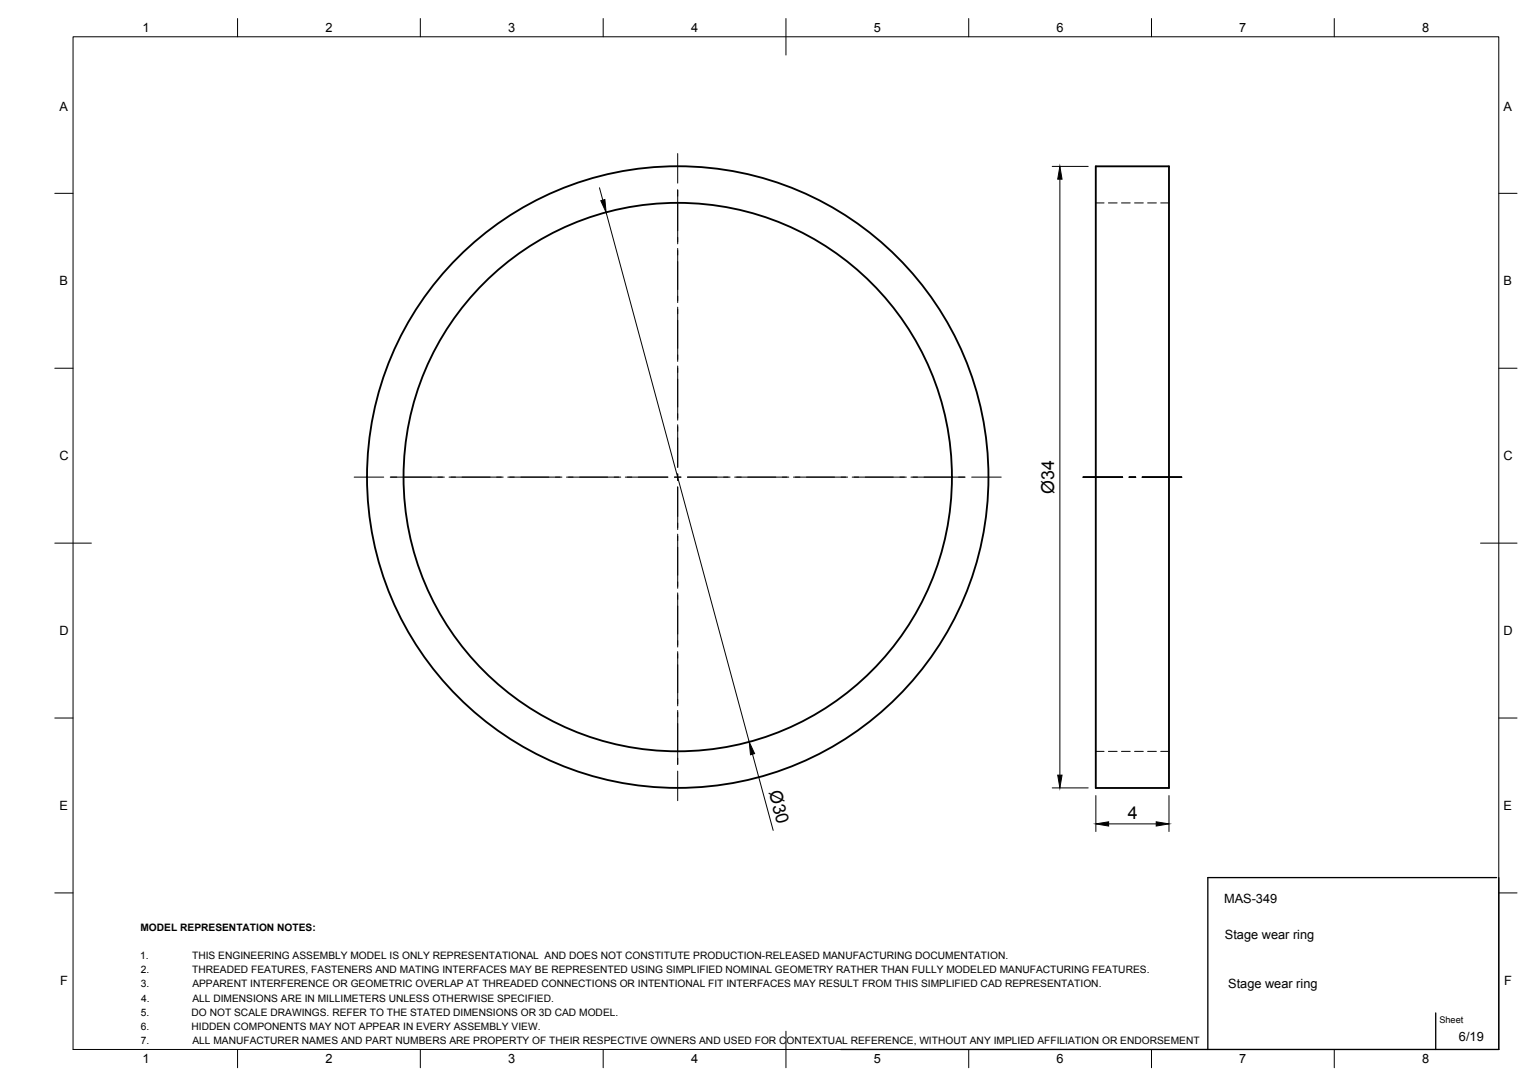
ISO-10303-21;
HEADER;
/* Generated by software containing ST-Developer
 * from STEP Tools, Inc. (www.steptools.com) 
 */

FILE_DESCRIPTION(
/* description */ ('Independent two-stage semi-open centrifugal-pump CAD. Shared impeller
s, open-machinable return casings, removable diaphragms, bronze wear/j
ournal rings, volume-preserving seal instances, retained keyed shaft, 
opposed mechanical face rings and partly threaded tie hardware. Native
 shaft rotation. Geometric topology/clearance only; flow/head/efficien
cy, pressure, cavitation, balance, preload, face loading and secondary
 seal fits/bonds, material/thermal/tolerance selection and life unassi
gned. External drive, coupling, anchors and piping bolts omitted.'),
/* implementation_level */ '2;1');

FILE_NAME(
/* name */ 'Stage wear ring.step',
/* time_stamp */ '2026-11-08T18:06:32-08:00',
/* author */ (''),
/* organization */ (''),
/* preprocessor_version */ 'ST-DEVELOPER v20.2',
/* originating_system */ 'Autodesk Translation Framework v15.17.0.0',
/* authorisation */ '');

FILE_SCHEMA (('AUTOMOTIVE_DESIGN { 1 0 10303 214 3 1 1 }'));
ENDSEC;

DATA;
#10=MECHANICAL_DESIGN_GEOMETRIC_PRESENTATION_REPRESENTATION('',(#396),#16687);
#358=SHAPE_REPRESENTATION_RELATIONSHIP('SRR','None',#16767,#377);
#377=ADVANCED_BREP_SHAPE_REPRESENTATION('',(#415),#16671);
#396=STYLED_ITEM('',(#16871),#415);
#415=MANIFOLD_SOLID_BREP('Body1',#6115);
#475=FACE_BOUND('',#1186,.T.);
#476=FACE_BOUND('',#1188,.T.);
#612=PLANE('',#6560);
#613=PLANE('',#6561);
#792=FACE_OUTER_BOUND('',#1183,.T.);
#793=FACE_OUTER_BOUND('',#1184,.T.);
#794=FACE_OUTER_BOUND('',#1185,.T.);
#795=FACE_OUTER_BOUND('',#1187,.T.);
#1183=EDGE_LOOP('',(#4395,#4396,#4397,#4398));
#1184=EDGE_LOOP('',(#4399,#4400,#4401,#4402));
#1185=EDGE_LOOP('',(#4403));
#1186=EDGE_LOOP('',(#4404));
#1187=EDGE_LOOP('',(#4405));
#1188=EDGE_LOOP('',(#4406));
#1652=LINE('',#9186,#2021);
#1653=LINE('',#9192,#2022);
#2021=VECTOR('',#7568,1.5);
#2022=VECTOR('',#7575,1.7);
#2342=CIRCLE('',#6555,1.5);
#2343=CIRCLE('',#6556,1.5);
#2344=CIRCLE('',#6558,1.7);
#2345=CIRCLE('',#6559,1.7);
#2667=VERTEX_POINT('',#9183);
#2668=VERTEX_POINT('',#9185);
#2669=VERTEX_POINT('',#9189);
#2670=VERTEX_POINT('',#9191);
#3307=EDGE_CURVE('',#2667,#2667,#2342,.T.);
#3308=EDGE_CURVE('',#2667,#2668,#1652,.T.);
#3309=EDGE_CURVE('',#2668,#2668,#2343,.T.);
#3310=EDGE_CURVE('',#2669,#2669,#2344,.T.);
#3311=EDGE_CURVE('',#2669,#2670,#1653,.T.);
#3312=EDGE_CURVE('',#2670,#2670,#2345,.T.);
#4395=ORIENTED_EDGE('',*,*,#3307,.F.);
#4396=ORIENTED_EDGE('',*,*,#3308,.T.);
#4397=ORIENTED_EDGE('',*,*,#3309,.T.);
#4398=ORIENTED_EDGE('',*,*,#3308,.F.);
#4399=ORIENTED_EDGE('',*,*,#3310,.F.);
#4400=ORIENTED_EDGE('',*,*,#3311,.T.);
#4401=ORIENTED_EDGE('',*,*,#3312,.T.);
#4402=ORIENTED_EDGE('',*,*,#3311,.F.);
#4403=ORIENTED_EDGE('',*,*,#3310,.T.);
#4404=ORIENTED_EDGE('',*,*,#3307,.T.);
#4405=ORIENTED_EDGE('',*,*,#3312,.F.);
#4406=ORIENTED_EDGE('',*,*,#3309,.F.);
#5610=CYLINDRICAL_SURFACE('',#6554,1.5);
#5611=CYLINDRICAL_SURFACE('',#6557,1.7);
#5871=ADVANCED_FACE('',(#792),#5610,.F.);
#5872=ADVANCED_FACE('',(#793),#5611,.T.);
#5873=ADVANCED_FACE('',(#794,#475),#612,.T.);
#5874=ADVANCED_FACE('',(#795,#476),#613,.F.);
#6115=CLOSED_SHELL('',(#5871,#5872,#5873,#5874));
#6553=AXIS2_PLACEMENT_3D('',#9181,#7562,#7563);
#6554=AXIS2_PLACEMENT_3D('',#9182,#7564,#7565);
#6555=AXIS2_PLACEMENT_3D('',#9184,#7566,#7567);
#6556=AXIS2_PLACEMENT_3D('',#9187,#7569,#7570);
#6557=AXIS2_PLACEMENT_3D('',#9188,#7571,#7572);
#6558=AXIS2_PLACEMENT_3D('',#9190,#7573,#7574);
#6559=AXIS2_PLACEMENT_3D('',#9193,#7576,#7577);
#6560=AXIS2_PLACEMENT_3D('',#9194,#7578,#7579);
#6561=AXIS2_PLACEMENT_3D('',#9195,#7580,#7581);
#7562=DIRECTION('axis',(0.,0.,1.));
#7563=DIRECTION('refdir',(1.,0.,0.));
#7564=DIRECTION('center_axis',(0.,0.,1.));
#7565=DIRECTION('ref_axis',(1.,0.,0.));
#7566=DIRECTION('center_axis',(0.,0.,-1.));
#7567=DIRECTION('ref_axis',(1.,0.,0.));
#7568=DIRECTION('',(0.,0.,-1.));
#7569=DIRECTION('center_axis',(0.,0.,-1.));
#7570=DIRECTION('ref_axis',(1.,0.,0.));
#7571=DIRECTION('center_axis',(0.,0.,1.));
#7572=DIRECTION('ref_axis',(1.,0.,0.));
#7573=DIRECTION('center_axis',(0.,0.,1.));
#7574=DIRECTION('ref_axis',(1.,0.,0.));
#7575=DIRECTION('',(0.,0.,-1.));
#7576=DIRECTION('center_axis',(0.,0.,1.));
#7577=DIRECTION('ref_axis',(1.,0.,0.));
#7578=DIRECTION('center_axis',(0.,0.,1.));
#7579=DIRECTION('ref_axis',(1.,0.,0.));
#7580=DIRECTION('center_axis',(0.,0.,1.));
#7581=DIRECTION('ref_axis',(1.,0.,0.));
#9181=CARTESIAN_POINT('',(0.,0.,0.));
#9182=CARTESIAN_POINT('Origin',(0.,0.,0.));
#9183=CARTESIAN_POINT('',(-1.5,-1.83697019872103E-16,0.4));
#9184=CARTESIAN_POINT('Origin',(0.,0.,0.4));
#9185=CARTESIAN_POINT('',(-1.5,-1.83697019872103E-16,0.));
#9186=CARTESIAN_POINT('',(-1.5,-1.83697019872103E-16,0.));
#9187=CARTESIAN_POINT('Origin',(0.,0.,0.));
#9188=CARTESIAN_POINT('Origin',(0.,0.,0.));
#9189=CARTESIAN_POINT('',(-1.7,-2.0818995585505E-16,0.4));
#9190=CARTESIAN_POINT('Origin',(0.,0.,0.4));
#9191=CARTESIAN_POINT('',(-1.7,-2.0818995585505E-16,0.));
#9192=CARTESIAN_POINT('',(-1.7,-2.0818995585505E-16,0.));
#9193=CARTESIAN_POINT('Origin',(0.,0.,0.));
#9194=CARTESIAN_POINT('Origin',(0.,0.,0.4));
#9195=CARTESIAN_POINT('Origin',(0.,0.,0.));
#16650=UNCERTAINTY_MEASURE_WITH_UNIT(LENGTH_MEASURE(0.001),#16688,
'DISTANCE_ACCURACY_VALUE',
'Maximum model space distance between geometric entities at asserted c
onnectivities');
#16666=UNCERTAINTY_MEASURE_WITH_UNIT(LENGTH_MEASURE(0.001),#16688,
'DISTANCE_ACCURACY_VALUE',
'Maximum model space distance between geometric entities at asserted c
onnectivities');
#16671=(
GEOMETRIC_REPRESENTATION_CONTEXT(3)
GLOBAL_UNCERTAINTY_ASSIGNED_CONTEXT((#16650))
GLOBAL_UNIT_ASSIGNED_CONTEXT((#16688,#16690,#16691))
REPRESENTATION_CONTEXT('','3D')
);
#16687=(
GEOMETRIC_REPRESENTATION_CONTEXT(3)
GLOBAL_UNCERTAINTY_ASSIGNED_CONTEXT((#16666))
GLOBAL_UNIT_ASSIGNED_CONTEXT((#16688,#16690,#16691))
REPRESENTATION_CONTEXT('','3D')
);
#16688=(
LENGTH_UNIT()
NAMED_UNIT(*)
SI_UNIT(.CENTI.,.METRE.)
);
#16690=(
NAMED_UNIT(*)
PLANE_ANGLE_UNIT()
SI_UNIT($,.RADIAN.)
);
#16691=(
NAMED_UNIT(*)
SI_UNIT($,.STERADIAN.)
SOLID_ANGLE_UNIT()
);
#16696=SHAPE_DEFINITION_REPRESENTATION(#16716,#16767);
#16716=PRODUCT_DEFINITION_SHAPE('',$,#16788);
#16767=SHAPE_REPRESENTATION('',(#6553),#16671);
#16783=PRODUCT_DEFINITION_CONTEXT('part definition',#16845,'design');
#16788=PRODUCT_DEFINITION('Stage wear ring','Stage wear ring',#16808,#16783);
#16808=PRODUCT_DEFINITION_FORMATION('',$,#16851);
#16845=APPLICATION_CONTEXT(
'Core Data for Automotive Mechanical Design Process');
#16846=PRODUCT_CONTEXT('part definition',#16845,'mechanical');
#16851=PRODUCT('Stage wear ring','Stage wear ring',$,(#16846));
#16871=PRESENTATION_STYLE_ASSIGNMENT((#16886));
#16886=SURFACE_STYLE_USAGE(.BOTH.,#16901);
#16901=SURFACE_SIDE_STYLE('',(#16916));
#16916=SURFACE_STYLE_FILL_AREA(#16931);
#16931=FILL_AREA_STYLE('Wear ring gray',(#16946));
#16946=FILL_AREA_STYLE_COLOUR('Wear ring gray',#16961);
#16961=COLOUR_RGB('Wear ring gray',0.725490196078431,0.752941176470588,
0.792156862745098);
ENDSEC;
END-ISO-10303-21;
